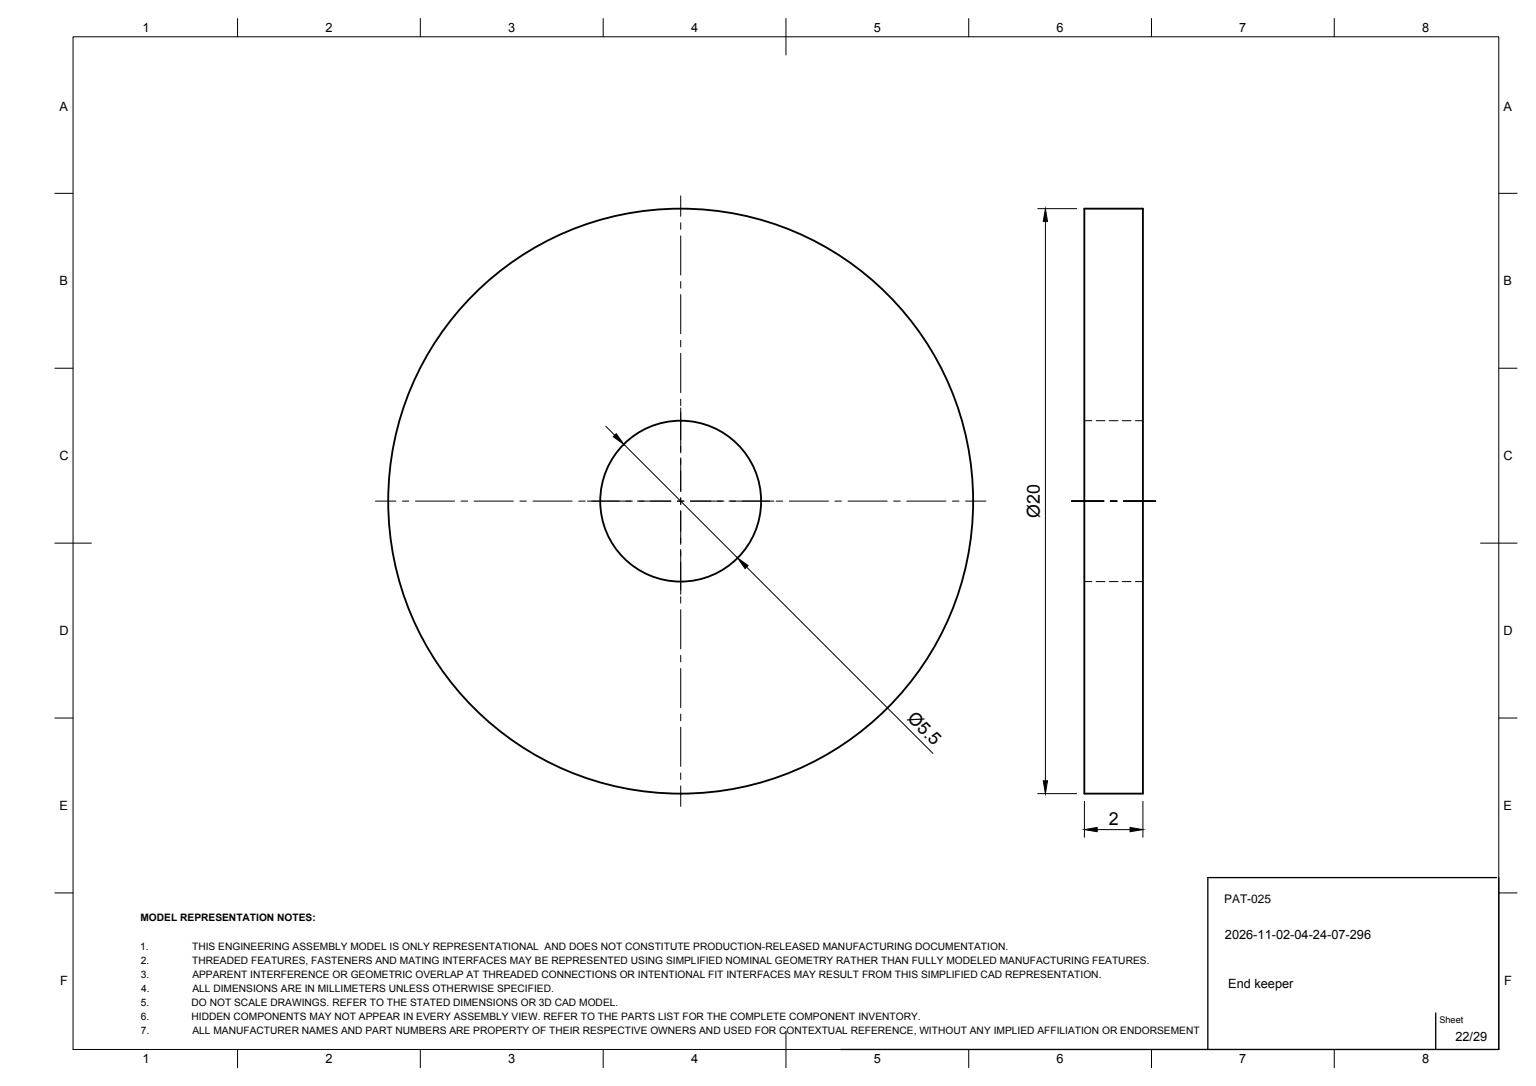
ISO-10303-21;
HEADER;
/* Generated by software containing ST-Developer
 * from STEP Tools, Inc. (www.steptools.com) 
 */

FILE_DESCRIPTION(
/* description */ ('Counter shaft with two pulleys and keyed hub'),
/* implementation_level */ '2;1');

FILE_NAME(
/* name */ 'End keeper.step',
/* time_stamp */ '2026-10-27T10:46:10-07:00',
/* author */ (''),
/* organization */ (''),
/* preprocessor_version */ 'ST-DEVELOPER v20.2',
/* originating_system */ 'Autodesk Translation Framework v15.17.0.0',
/* authorisation */ '');

FILE_SCHEMA (('AUTOMOTIVE_DESIGN { 1 0 10303 214 3 1 1 }'));
ENDSEC;

DATA;
#10=MECHANICAL_DESIGN_GEOMETRIC_PRESENTATION_REPRESENTATION('',(#306),#10821);
#255=SHAPE_REPRESENTATION_RELATIONSHIP('SRR','None',#10943,#280);
#280=ADVANCED_BREP_SHAPE_REPRESENTATION('',(#331),#10811);
#306=STYLED_ITEM('',(#11149),#331);
#331=MANIFOLD_SOLID_BREP('Body1',#5590);
#401=FACE_BOUND('',#1103,.T.);
#402=FACE_BOUND('',#1105,.T.);
#521=PLANE('',#6148);
#522=PLANE('',#6149);
#725=FACE_OUTER_BOUND('',#1100,.T.);
#726=FACE_OUTER_BOUND('',#1101,.T.);
#727=FACE_OUTER_BOUND('',#1102,.T.);
#728=FACE_OUTER_BOUND('',#1104,.T.);
#1100=EDGE_LOOP('',(#4195,#4196,#4197,#4198));
#1101=EDGE_LOOP('',(#4199,#4200,#4201,#4202));
#1102=EDGE_LOOP('',(#4203));
#1103=EDGE_LOOP('',(#4204));
#1104=EDGE_LOOP('',(#4205));
#1105=EDGE_LOOP('',(#4206));
#1477=LINE('',#9378,#1866);
#1478=LINE('',#9384,#1867);
#1866=VECTOR('',#7263,0.275);
#1867=VECTOR('',#7270,1.);
#2174=CIRCLE('',#6143,0.275);
#2175=CIRCLE('',#6144,0.275);
#2176=CIRCLE('',#6146,1.);
#2177=CIRCLE('',#6147,1.);
#2579=VERTEX_POINT('',#9375);
#2580=VERTEX_POINT('',#9377);
#2581=VERTEX_POINT('',#9381);
#2582=VERTEX_POINT('',#9383);
#3170=EDGE_CURVE('',#2579,#2579,#2174,.T.);
#3171=EDGE_CURVE('',#2579,#2580,#1477,.T.);
#3172=EDGE_CURVE('',#2580,#2580,#2175,.T.);
#3173=EDGE_CURVE('',#2581,#2581,#2176,.T.);
#3174=EDGE_CURVE('',#2581,#2582,#1478,.T.);
#3175=EDGE_CURVE('',#2582,#2582,#2177,.T.);
#4195=ORIENTED_EDGE('',*,*,#3170,.F.);
#4196=ORIENTED_EDGE('',*,*,#3171,.T.);
#4197=ORIENTED_EDGE('',*,*,#3172,.T.);
#4198=ORIENTED_EDGE('',*,*,#3171,.F.);
#4199=ORIENTED_EDGE('',*,*,#3173,.F.);
#4200=ORIENTED_EDGE('',*,*,#3174,.T.);
#4201=ORIENTED_EDGE('',*,*,#3175,.T.);
#4202=ORIENTED_EDGE('',*,*,#3174,.F.);
#4203=ORIENTED_EDGE('',*,*,#3173,.T.);
#4204=ORIENTED_EDGE('',*,*,#3170,.T.);
#4205=ORIENTED_EDGE('',*,*,#3175,.F.);
#4206=ORIENTED_EDGE('',*,*,#3172,.F.);
#5155=CYLINDRICAL_SURFACE('',#6142,0.275);
#5156=CYLINDRICAL_SURFACE('',#6145,1.);
#5396=ADVANCED_FACE('',(#725),#5155,.F.);
#5397=ADVANCED_FACE('',(#726),#5156,.T.);
#5398=ADVANCED_FACE('',(#727,#401),#521,.T.);
#5399=ADVANCED_FACE('',(#728,#402),#522,.F.);
#5590=CLOSED_SHELL('',(#5396,#5397,#5398,#5399));
#6141=AXIS2_PLACEMENT_3D('',#9373,#7257,#7258);
#6142=AXIS2_PLACEMENT_3D('',#9374,#7259,#7260);
#6143=AXIS2_PLACEMENT_3D('',#9376,#7261,#7262);
#6144=AXIS2_PLACEMENT_3D('',#9379,#7264,#7265);
#6145=AXIS2_PLACEMENT_3D('',#9380,#7266,#7267);
#6146=AXIS2_PLACEMENT_3D('',#9382,#7268,#7269);
#6147=AXIS2_PLACEMENT_3D('',#9385,#7271,#7272);
#6148=AXIS2_PLACEMENT_3D('',#9386,#7273,#7274);
#6149=AXIS2_PLACEMENT_3D('',#9387,#7275,#7276);
#7257=DIRECTION('axis',(0.,0.,1.));
#7258=DIRECTION('refdir',(1.,0.,0.));
#7259=DIRECTION('center_axis',(0.,1.,0.));
#7260=DIRECTION('ref_axis',(1.,0.,0.));
#7261=DIRECTION('center_axis',(0.,-1.,0.));
#7262=DIRECTION('ref_axis',(1.,0.,0.));
#7263=DIRECTION('',(0.,-1.,0.));
#7264=DIRECTION('center_axis',(0.,-1.,0.));
#7265=DIRECTION('ref_axis',(1.,0.,0.));
#7266=DIRECTION('center_axis',(0.,1.,0.));
#7267=DIRECTION('ref_axis',(1.,0.,0.));
#7268=DIRECTION('center_axis',(0.,1.,0.));
#7269=DIRECTION('ref_axis',(1.,0.,0.));
#7270=DIRECTION('',(0.,-1.,0.));
#7271=DIRECTION('center_axis',(0.,1.,0.));
#7272=DIRECTION('ref_axis',(1.,0.,0.));
#7273=DIRECTION('center_axis',(0.,1.,0.));
#7274=DIRECTION('ref_axis',(1.,0.,0.));
#7275=DIRECTION('center_axis',(0.,1.,0.));
#7276=DIRECTION('ref_axis',(1.,0.,0.));
#9373=CARTESIAN_POINT('',(0.,0.,0.));
#9374=CARTESIAN_POINT('Origin',(0.,-5.7,4.53));
#9375=CARTESIAN_POINT('',(-0.275,-5.5,4.53));
#9376=CARTESIAN_POINT('Origin',(0.,-5.5,4.53));
#9377=CARTESIAN_POINT('',(-0.275,-5.7,4.53));
#9378=CARTESIAN_POINT('',(-0.275,-5.7,4.53));
#9379=CARTESIAN_POINT('Origin',(0.,-5.7,4.53));
#9380=CARTESIAN_POINT('Origin',(0.,-5.7,4.53));
#9381=CARTESIAN_POINT('',(-1.,-5.5,4.53));
#9382=CARTESIAN_POINT('Origin',(0.,-5.5,4.53));
#9383=CARTESIAN_POINT('',(-1.,-5.7,4.53));
#9384=CARTESIAN_POINT('',(-1.,-5.7,4.53));
#9385=CARTESIAN_POINT('Origin',(0.,-5.7,4.53));
#9386=CARTESIAN_POINT('Origin',(0.,-5.5,4.53));
#9387=CARTESIAN_POINT('Origin',(0.,-5.7,4.53));
#10781=UNCERTAINTY_MEASURE_WITH_UNIT(LENGTH_MEASURE(0.001),#10822,
'DISTANCE_ACCURACY_VALUE',
'Maximum model space distance between geometric entities at asserted c
onnectivities');
#10791=UNCERTAINTY_MEASURE_WITH_UNIT(LENGTH_MEASURE(0.001),#10822,
'DISTANCE_ACCURACY_VALUE',
'Maximum model space distance between geometric entities at asserted c
onnectivities');
#10811=(
GEOMETRIC_REPRESENTATION_CONTEXT(3)
GLOBAL_UNCERTAINTY_ASSIGNED_CONTEXT((#10781))
GLOBAL_UNIT_ASSIGNED_CONTEXT((#10822,#10824,#10825))
REPRESENTATION_CONTEXT('','3D')
);
#10821=(
GEOMETRIC_REPRESENTATION_CONTEXT(3)
GLOBAL_UNCERTAINTY_ASSIGNED_CONTEXT((#10791))
GLOBAL_UNIT_ASSIGNED_CONTEXT((#10822,#10824,#10825))
REPRESENTATION_CONTEXT('','3D')
);
#10822=(
LENGTH_UNIT()
NAMED_UNIT(*)
SI_UNIT(.CENTI.,.METRE.)
);
#10824=(
NAMED_UNIT(*)
PLANE_ANGLE_UNIT()
SI_UNIT($,.RADIAN.)
);
#10825=(
NAMED_UNIT(*)
SI_UNIT($,.STERADIAN.)
SOLID_ANGLE_UNIT()
);
#10845=SHAPE_DEFINITION_REPRESENTATION(#10893,#10943);
#10893=PRODUCT_DEFINITION_SHAPE('',$,#10973);
#10943=SHAPE_REPRESENTATION('',(#6141),#10811);
#10953=PRODUCT_DEFINITION_CONTEXT('part definition',#11042,'design');
#10973=PRODUCT_DEFINITION('End keeper','End keeper',#11002,#10953);
#11002=PRODUCT_DEFINITION_FORMATION('',$,#11063);
#11042=APPLICATION_CONTEXT(
'Core Data for Automotive Mechanical Design Process');
#11043=PRODUCT_CONTEXT('part definition',#11042,'mechanical');
#11063=PRODUCT('End keeper','End keeper','End keeper',(#11043));
#11143=COLOUR_RGB('Off White',0.89,0.88,0.83);
#11144=FILL_AREA_STYLE_COLOUR('',#11143);
#11145=FILL_AREA_STYLE('',(#11144));
#11146=SURFACE_STYLE_FILL_AREA(#11145);
#11147=SURFACE_SIDE_STYLE('',(#11146));
#11148=SURFACE_STYLE_USAGE(.BOTH.,#11147);
#11149=PRESENTATION_STYLE_ASSIGNMENT((#11148));
ENDSEC;
END-ISO-10303-21;
